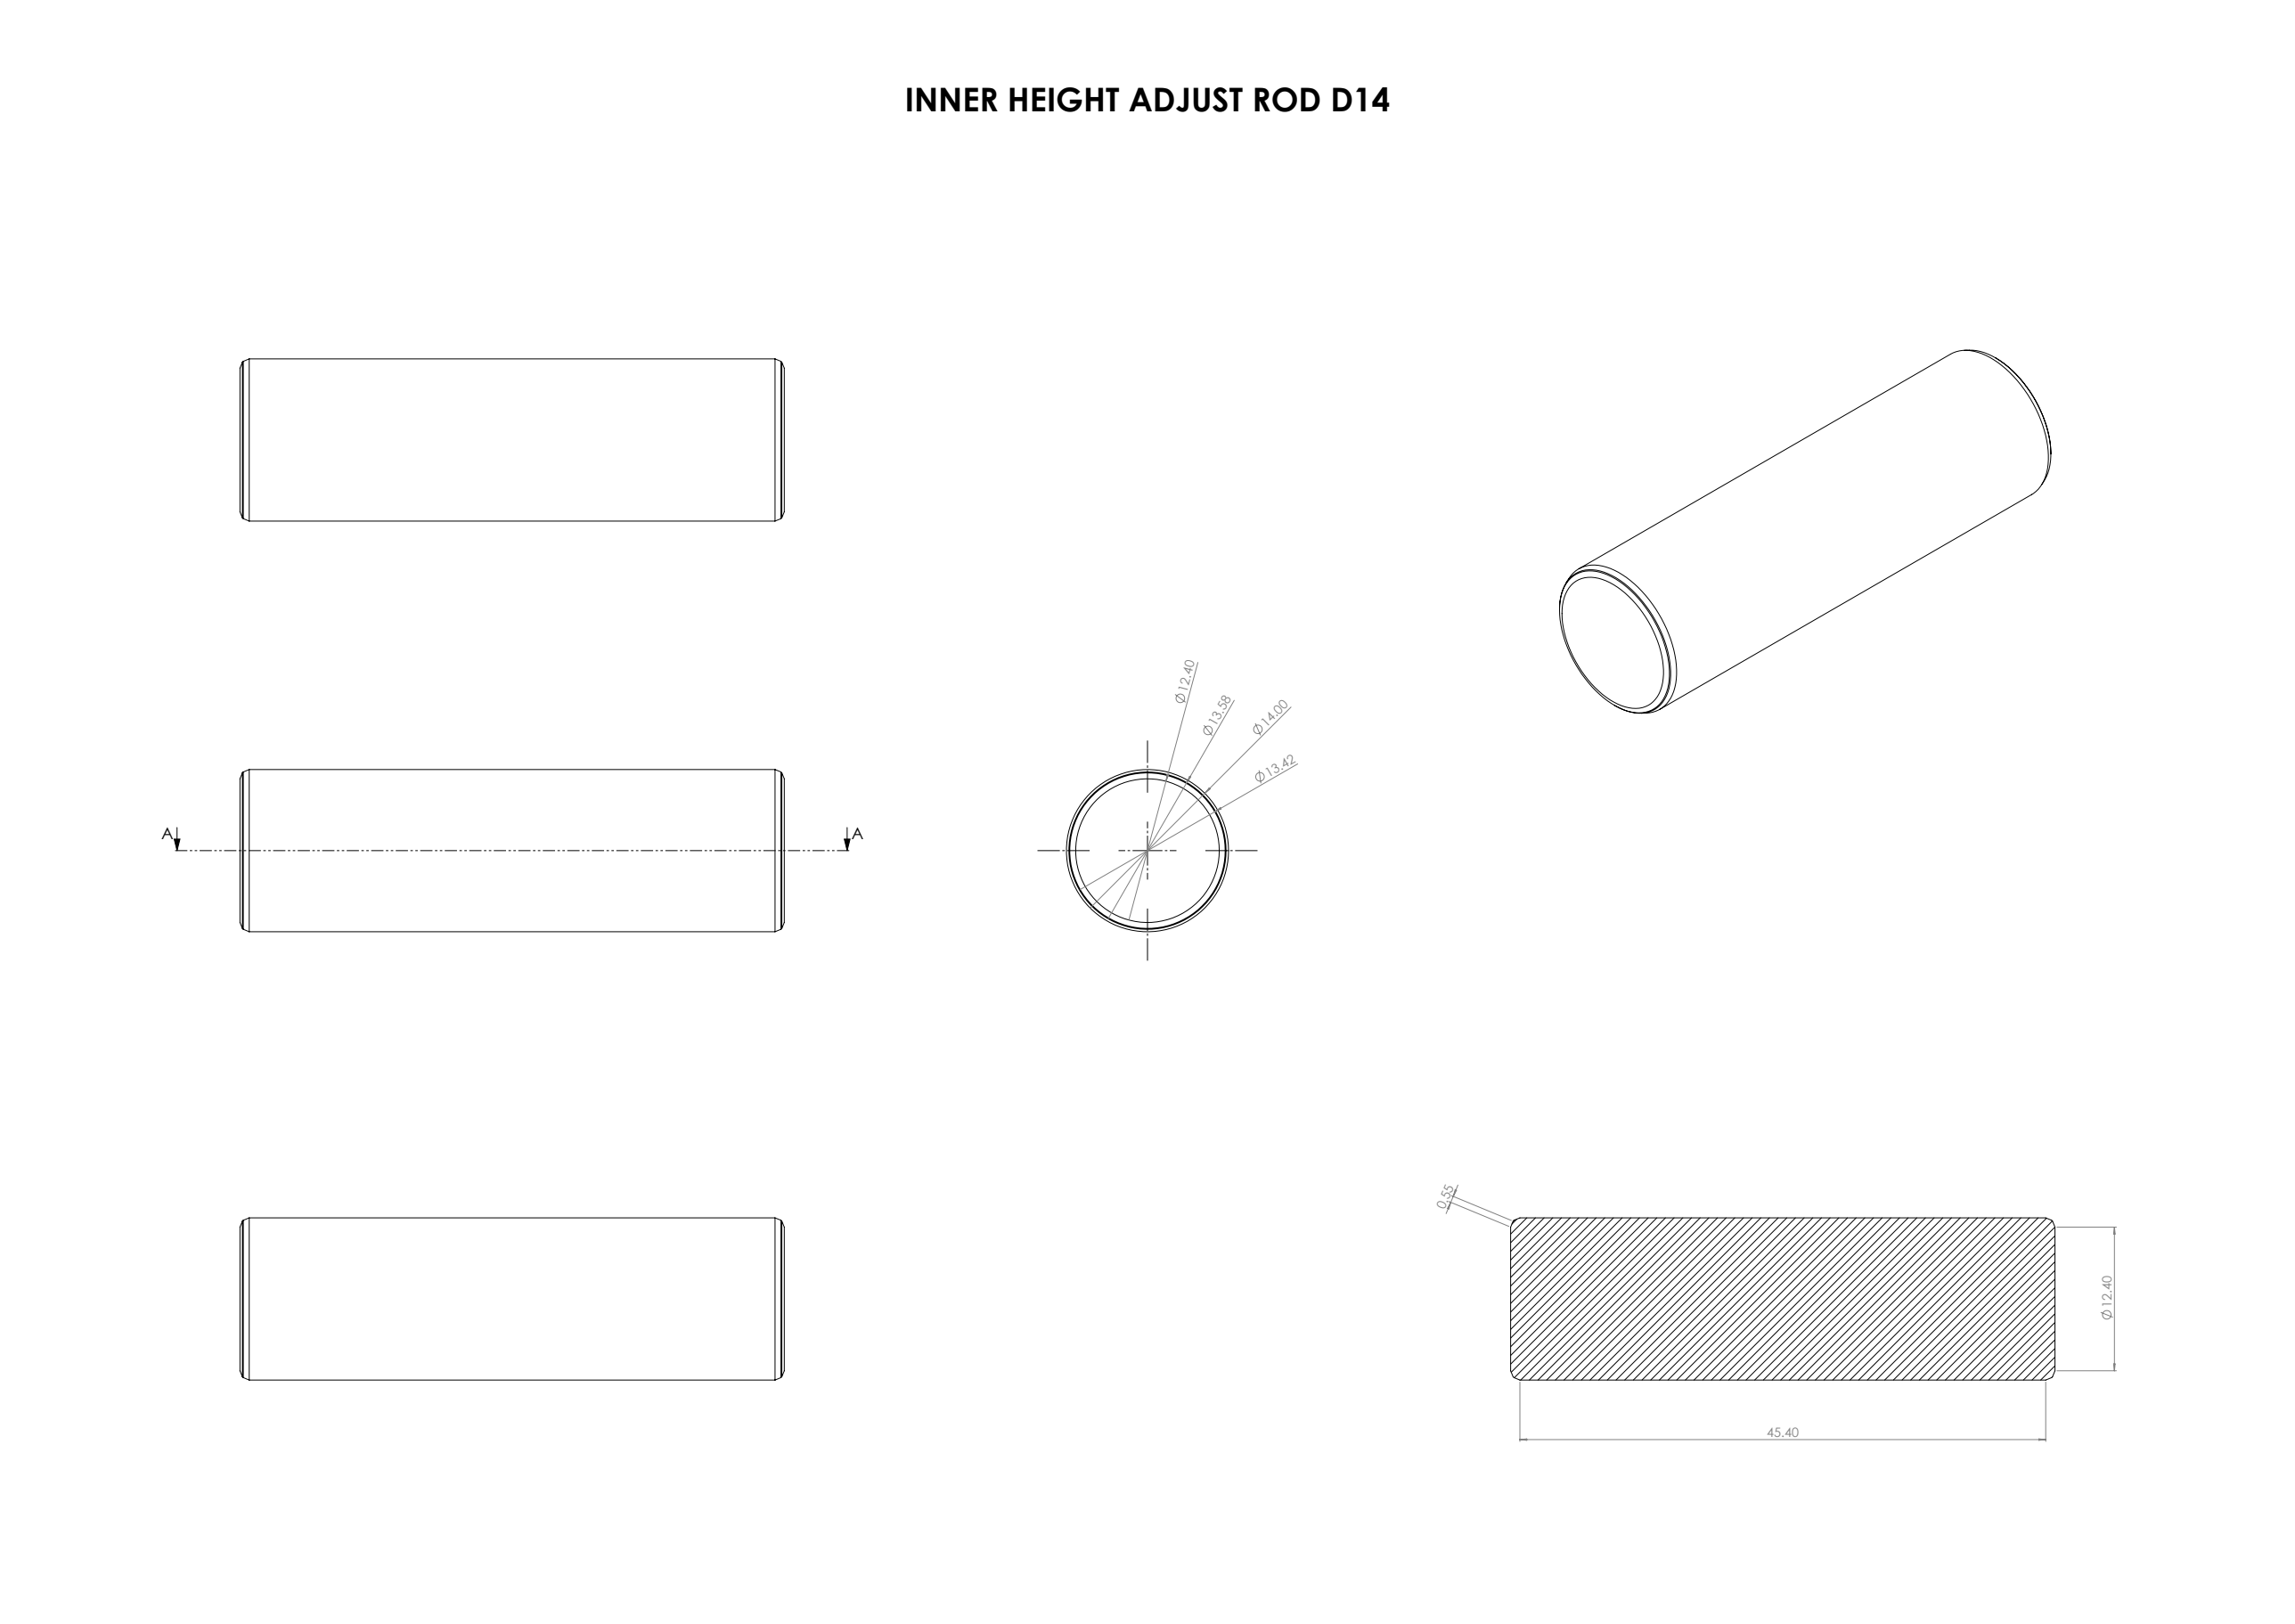
ISO-10303-21;
HEADER;
/* Generated by software containing ST-Developer
 * from STEP Tools, Inc. (www.steptools.com) 
 */

FILE_DESCRIPTION(
/* description */ (''),
/* implementation_level */ '2;1');

FILE_NAME(
/* name */ 
'03_Inner_Height_Adjust_Rod_D14.step',
/* time_stamp */ '2026-10-20T10:06:23-07:00',
/* author */ (''),
/* organization */ (''),
/* preprocessor_version */ 'ST-DEVELOPER v20.2',
/* originating_system */ 'Autodesk Translation Framework v15.15.0.0',
/* authorisation */ '');

FILE_SCHEMA (('AUTOMOTIVE_DESIGN { 1 0 10303 214 3 1 1 }'));
ENDSEC;

DATA;
#10=MECHANICAL_DESIGN_GEOMETRIC_PRESENTATION_REPRESENTATION('',(#462),#38611);
#434=SHAPE_REPRESENTATION_RELATIONSHIP('SRR','None',#38670,#448);
#448=ADVANCED_BREP_SHAPE_REPRESENTATION('',(#476),#38599);
#462=STYLED_ITEM('',(#38878),#476);
#476=MANIFOLD_SOLID_BREP('Rod',#16236);
#895=CYLINDRICAL_SURFACE('',#16637,0.7);
#1279=CIRCLE('',#16627,0.619999999999999);
#1280=CIRCLE('',#16628,0.671213203435596);
#1281=CIRCLE('',#16629,0.671213203435596);
#1282=CIRCLE('',#16631,0.678786796564404);
#1283=CIRCLE('',#16632,0.678786796564404);
#1284=CIRCLE('',#16635,0.7);
#1285=CIRCLE('',#16636,0.7);
#1286=CIRCLE('',#16638,0.7);
#1287=CIRCLE('',#16639,0.7);
#1288=CIRCLE('',#16641,0.678786796564404);
#1289=CIRCLE('',#16642,0.678786796564404);
#1290=CIRCLE('',#16644,0.671213203435597);
#1291=CIRCLE('',#16645,0.671213203435597);
#1292=CIRCLE('',#16647,0.62);
#1709=CONICAL_SURFACE('',#16626,0.645606601717798,1.17809724509618);
#1710=CONICAL_SURFACE('',#16630,0.675,0.78539816339745);
#1711=CONICAL_SURFACE('',#16634,0.689393398282202,0.392699081698726);
#1712=CONICAL_SURFACE('',#16640,0.689393398282202,0.392699081698718);
#1713=CONICAL_SURFACE('',#16643,0.675,0.785398163397447);
#1714=CONICAL_SURFACE('',#16646,0.645606601717798,1.17809724509617);
#1921=FACE_OUTER_BOUND('',#2848,.T.);
#1922=FACE_OUTER_BOUND('',#2849,.T.);
#1923=FACE_OUTER_BOUND('',#2850,.T.);
#1924=FACE_OUTER_BOUND('',#2851,.T.);
#1925=FACE_OUTER_BOUND('',#2852,.T.);
#1926=FACE_OUTER_BOUND('',#2853,.T.);
#1927=FACE_OUTER_BOUND('',#2854,.T.);
#1928=FACE_OUTER_BOUND('',#2855,.T.);
#1929=FACE_OUTER_BOUND('',#2856,.T.);
#2848=EDGE_LOOP('',(#10711,#10712,#10713,#10714,#10715));
#2849=EDGE_LOOP('',(#10716,#10717,#10718,#10719,#10720,#10721));
#2850=EDGE_LOOP('',(#10722));
#2851=EDGE_LOOP('',(#10723,#10724,#10725,#10726,#10727,#10728));
#2852=EDGE_LOOP('',(#10729,#10730,#10731,#10732,#10733,#10734));
#2853=EDGE_LOOP('',(#10735,#10736,#10737,#10738,#10739,#10740));
#2854=EDGE_LOOP('',(#10741,#10742,#10743,#10744,#10745,#10746));
#2855=EDGE_LOOP('',(#10747,#10748,#10749,#10750,#10751));
#2856=EDGE_LOOP('',(#10752));
#3908=LINE('',#22921,#5132);
#3909=LINE('',#22927,#5133);
#3910=LINE('',#22934,#5134);
#3911=LINE('',#22940,#5135);
#3912=LINE('',#22946,#5136);
#3913=LINE('',#22952,#5137);
#3914=LINE('',#22958,#5138);
#5132=VECTOR('',#18509,0.645606601717798);
#5133=VECTOR('',#18516,0.675);
#5134=VECTOR('',#18525,0.689393398282202);
#5135=VECTOR('',#18532,0.7);
#5136=VECTOR('',#18539,0.689393398282202);
#5137=VECTOR('',#18546,0.675);
#5138=VECTOR('',#18553,0.645606601717798);
#6309=VERTEX_POINT('',#22918);
#6310=VERTEX_POINT('',#22920);
#6311=VERTEX_POINT('',#22922);
#6312=VERTEX_POINT('',#22926);
#6313=VERTEX_POINT('',#22928);
#6314=VERTEX_POINT('',#22933);
#6315=VERTEX_POINT('',#22935);
#6316=VERTEX_POINT('',#22939);
#6317=VERTEX_POINT('',#22941);
#6318=VERTEX_POINT('',#22945);
#6319=VERTEX_POINT('',#22947);
#6320=VERTEX_POINT('',#22951);
#6321=VERTEX_POINT('',#22953);
#6322=VERTEX_POINT('',#22957);
#7971=EDGE_CURVE('',#6309,#6309,#1279,.T.);
#7972=EDGE_CURVE('',#6309,#6310,#3908,.T.);
#7973=EDGE_CURVE('',#6310,#6311,#1280,.T.);
#7974=EDGE_CURVE('',#6311,#6310,#1281,.T.);
#7975=EDGE_CURVE('',#6311,#6312,#3909,.T.);
#7976=EDGE_CURVE('',#6313,#6312,#1282,.T.);
#7977=EDGE_CURVE('',#6312,#6313,#1283,.T.);
#7978=EDGE_CURVE('',#6313,#6314,#3910,.T.);
#7979=EDGE_CURVE('',#6314,#6315,#1284,.T.);
#7980=EDGE_CURVE('',#6315,#6314,#1285,.T.);
#7981=EDGE_CURVE('',#6315,#6316,#3911,.T.);
#7982=EDGE_CURVE('',#6317,#6316,#1286,.T.);
#7983=EDGE_CURVE('',#6316,#6317,#1287,.T.);
#7984=EDGE_CURVE('',#6317,#6318,#3912,.T.);
#7985=EDGE_CURVE('',#6318,#6319,#1288,.T.);
#7986=EDGE_CURVE('',#6319,#6318,#1289,.T.);
#7987=EDGE_CURVE('',#6319,#6320,#3913,.T.);
#7988=EDGE_CURVE('',#6321,#6320,#1290,.T.);
#7989=EDGE_CURVE('',#6320,#6321,#1291,.T.);
#7990=EDGE_CURVE('',#6321,#6322,#3914,.T.);
#7991=EDGE_CURVE('',#6322,#6322,#1292,.T.);
#10711=ORIENTED_EDGE('',*,*,#7971,.T.);
#10712=ORIENTED_EDGE('',*,*,#7972,.T.);
#10713=ORIENTED_EDGE('',*,*,#7973,.T.);
#10714=ORIENTED_EDGE('',*,*,#7974,.T.);
#10715=ORIENTED_EDGE('',*,*,#7972,.F.);
#10716=ORIENTED_EDGE('',*,*,#7973,.F.);
#10717=ORIENTED_EDGE('',*,*,#7974,.F.);
#10718=ORIENTED_EDGE('',*,*,#7975,.T.);
#10719=ORIENTED_EDGE('',*,*,#7976,.F.);
#10720=ORIENTED_EDGE('',*,*,#7977,.F.);
#10721=ORIENTED_EDGE('',*,*,#7975,.F.);
#10722=ORIENTED_EDGE('',*,*,#7971,.F.);
#10723=ORIENTED_EDGE('',*,*,#7976,.T.);
#10724=ORIENTED_EDGE('',*,*,#7977,.T.);
#10725=ORIENTED_EDGE('',*,*,#7978,.T.);
#10726=ORIENTED_EDGE('',*,*,#7979,.T.);
#10727=ORIENTED_EDGE('',*,*,#7980,.T.);
#10728=ORIENTED_EDGE('',*,*,#7978,.F.);
#10729=ORIENTED_EDGE('',*,*,#7979,.F.);
#10730=ORIENTED_EDGE('',*,*,#7980,.F.);
#10731=ORIENTED_EDGE('',*,*,#7981,.T.);
#10732=ORIENTED_EDGE('',*,*,#7982,.F.);
#10733=ORIENTED_EDGE('',*,*,#7983,.F.);
#10734=ORIENTED_EDGE('',*,*,#7981,.F.);
#10735=ORIENTED_EDGE('',*,*,#7982,.T.);
#10736=ORIENTED_EDGE('',*,*,#7983,.T.);
#10737=ORIENTED_EDGE('',*,*,#7984,.T.);
#10738=ORIENTED_EDGE('',*,*,#7985,.T.);
#10739=ORIENTED_EDGE('',*,*,#7986,.T.);
#10740=ORIENTED_EDGE('',*,*,#7984,.F.);
#10741=ORIENTED_EDGE('',*,*,#7985,.F.);
#10742=ORIENTED_EDGE('',*,*,#7986,.F.);
#10743=ORIENTED_EDGE('',*,*,#7987,.T.);
#10744=ORIENTED_EDGE('',*,*,#7988,.F.);
#10745=ORIENTED_EDGE('',*,*,#7989,.F.);
#10746=ORIENTED_EDGE('',*,*,#7987,.F.);
#10747=ORIENTED_EDGE('',*,*,#7988,.T.);
#10748=ORIENTED_EDGE('',*,*,#7989,.T.);
#10749=ORIENTED_EDGE('',*,*,#7990,.T.);
#10750=ORIENTED_EDGE('',*,*,#7991,.T.);
#10751=ORIENTED_EDGE('',*,*,#7990,.F.);
#10752=ORIENTED_EDGE('',*,*,#7991,.F.);
#14896=PLANE('',#16633);
#14897=PLANE('',#16648);
#15464=ADVANCED_FACE('',(#1921),#1709,.T.);
#15465=ADVANCED_FACE('',(#1922),#1710,.T.);
#15466=ADVANCED_FACE('',(#1923),#14896,.T.);
#15467=ADVANCED_FACE('',(#1924),#1711,.T.);
#15468=ADVANCED_FACE('',(#1925),#895,.T.);
#15469=ADVANCED_FACE('',(#1926),#1712,.T.);
#15470=ADVANCED_FACE('',(#1927),#1713,.T.);
#15471=ADVANCED_FACE('',(#1928),#1714,.T.);
#15472=ADVANCED_FACE('',(#1929),#14897,.T.);
#16236=CLOSED_SHELL('',(#15464,#15465,#15466,#15467,#15468,#15469,#15470,
#15471,#15472));
#16625=AXIS2_PLACEMENT_3D('',#22916,#18503,#18504);
#16626=AXIS2_PLACEMENT_3D('',#22917,#18505,#18506);
#16627=AXIS2_PLACEMENT_3D('',#22919,#18507,#18508);
#16628=AXIS2_PLACEMENT_3D('',#22923,#18510,#18511);
#16629=AXIS2_PLACEMENT_3D('',#22924,#18512,#18513);
#16630=AXIS2_PLACEMENT_3D('',#22925,#18514,#18515);
#16631=AXIS2_PLACEMENT_3D('',#22929,#18517,#18518);
#16632=AXIS2_PLACEMENT_3D('',#22930,#18519,#18520);
#16633=AXIS2_PLACEMENT_3D('',#22931,#18521,#18522);
#16634=AXIS2_PLACEMENT_3D('',#22932,#18523,#18524);
#16635=AXIS2_PLACEMENT_3D('',#22936,#18526,#18527);
#16636=AXIS2_PLACEMENT_3D('',#22937,#18528,#18529);
#16637=AXIS2_PLACEMENT_3D('',#22938,#18530,#18531);
#16638=AXIS2_PLACEMENT_3D('',#22942,#18533,#18534);
#16639=AXIS2_PLACEMENT_3D('',#22943,#18535,#18536);
#16640=AXIS2_PLACEMENT_3D('',#22944,#18537,#18538);
#16641=AXIS2_PLACEMENT_3D('',#22948,#18540,#18541);
#16642=AXIS2_PLACEMENT_3D('',#22949,#18542,#18543);
#16643=AXIS2_PLACEMENT_3D('',#22950,#18544,#18545);
#16644=AXIS2_PLACEMENT_3D('',#22954,#18547,#18548);
#16645=AXIS2_PLACEMENT_3D('',#22955,#18549,#18550);
#16646=AXIS2_PLACEMENT_3D('',#22956,#18551,#18552);
#16647=AXIS2_PLACEMENT_3D('',#22959,#18554,#18555);
#16648=AXIS2_PLACEMENT_3D('',#22960,#18556,#18557);
#18503=DIRECTION('axis',(0.,0.,1.));
#18504=DIRECTION('refdir',(1.,0.,0.));
#18505=DIRECTION('center_axis',(0.,-1.93747046180099E-15,-1.));
#18506=DIRECTION('ref_axis',(-1.,-3.18304947217744E-17,0.));
#18507=DIRECTION('center_axis',(0.,0.,-1.));
#18508=DIRECTION('ref_axis',(-1.,0.,0.));
#18509=DIRECTION('',(0.923879532511291,-5.98887692616032E-16,-0.38268343236508));
#18510=DIRECTION('center_axis',(0.,0.,1.));
#18511=DIRECTION('ref_axis',(-1.,-6.12323399573677E-17,0.));
#18512=DIRECTION('center_axis',(0.,0.,1.));
#18513=DIRECTION('ref_axis',(-1.,-6.12323399573677E-17,0.));
#18514=DIRECTION('center_axis',(0.,0.,-1.));
#18515=DIRECTION('ref_axis',(1.,0.,0.));
#18516=DIRECTION('',(-0.707106781186548,-8.65956056235494E-17,-0.707106781186547));
#18517=DIRECTION('center_axis',(0.,0.,-1.));
#18518=DIRECTION('ref_axis',(-1.,-6.12323399573677E-17,0.));
#18519=DIRECTION('center_axis',(0.,0.,-1.));
#18520=DIRECTION('ref_axis',(-1.,-6.12323399573677E-17,0.));
#18521=DIRECTION('center_axis',(0.,0.,1.));
#18522=DIRECTION('ref_axis',(1.,0.,0.));
#18523=DIRECTION('center_axis',(0.,8.11581801128163E-16,-1.));
#18524=DIRECTION('ref_axis',(-1.,-3.01451275783686E-17,0.));
#18525=DIRECTION('',(0.382683432365092,8.08205059964992E-16,-0.923879532511286));
#18526=DIRECTION('center_axis',(0.,0.,1.));
#18527=DIRECTION('ref_axis',(-1.,0.,0.));
#18528=DIRECTION('center_axis',(0.,0.,1.));
#18529=DIRECTION('ref_axis',(-1.,0.,0.));
#18530=DIRECTION('center_axis',(0.,0.,1.));
#18531=DIRECTION('ref_axis',(1.,0.,0.));
#18532=DIRECTION('',(0.,0.,-1.));
#18533=DIRECTION('center_axis',(0.,0.,-1.));
#18534=DIRECTION('ref_axis',(-1.,0.,0.));
#18535=DIRECTION('center_axis',(0.,0.,-1.));
#18536=DIRECTION('ref_axis',(-1.,0.,0.));
#18537=DIRECTION('center_axis',(0.,8.11581801128149E-16,1.));
#18538=DIRECTION('ref_axis',(-1.,-3.01451275783686E-17,0.));
#18539=DIRECTION('',(-0.382683432365084,-8.0820505996498E-16,-0.923879532511289));
#18540=DIRECTION('center_axis',(0.,0.,1.));
#18541=DIRECTION('ref_axis',(-1.,-6.12323399573677E-17,0.));
#18542=DIRECTION('center_axis',(0.,0.,1.));
#18543=DIRECTION('ref_axis',(-1.,-6.12323399573677E-17,0.));
#18544=DIRECTION('center_axis',(0.,0.,1.));
#18545=DIRECTION('ref_axis',(1.,0.,0.));
#18546=DIRECTION('',(0.707106781186547,8.65956056235492E-17,-0.707106781186548));
#18547=DIRECTION('center_axis',(0.,0.,-1.));
#18548=DIRECTION('ref_axis',(-1.,-6.12323399573676E-17,0.));
#18549=DIRECTION('center_axis',(0.,0.,-1.));
#18550=DIRECTION('ref_axis',(-1.,-6.12323399573676E-17,0.));
#18551=DIRECTION('center_axis',(0.,-1.93747046180093E-15,1.));
#18552=DIRECTION('ref_axis',(-1.,-3.18304947217744E-17,0.));
#18553=DIRECTION('',(-0.923879532511287,5.98887692616029E-16,-0.38268343236509));
#18554=DIRECTION('center_axis',(0.,0.,1.));
#18555=DIRECTION('ref_axis',(-1.,0.,0.));
#18556=DIRECTION('center_axis',(0.,0.,-1.));
#18557=DIRECTION('ref_axis',(-1.,0.,0.));
#22916=CARTESIAN_POINT('',(0.,0.,0.));
#22917=CARTESIAN_POINT('Origin',(0.,-2.05499775283211E-17,6.0893933982822));
#22918=CARTESIAN_POINT('',(0.619999999999999,-7.59281015471358E-17,6.1));
#22919=CARTESIAN_POINT('Origin',(0.,0.,6.1));
#22920=CARTESIAN_POINT('',(0.671213203435596,8.21999101132844E-17,6.0787867965644));
#22921=CARTESIAN_POINT('',(0.645606601717798,7.90640058302101E-17,6.0893933982822));
#22922=CARTESIAN_POINT('',(-0.671213203435596,-8.21999101132843E-17,6.0787867965644));
#22923=CARTESIAN_POINT('Origin',(0.,-4.10999550566422E-17,6.0787867965644));
#22924=CARTESIAN_POINT('Origin',(0.,-4.10999550566422E-17,6.0787867965644));
#22925=CARTESIAN_POINT('Origin',(0.,0.,6.075));
#22926=CARTESIAN_POINT('',(-0.678786796564404,-8.31274077716083E-17,6.0712132034356));
#22927=CARTESIAN_POINT('',(-0.675,-8.26636589424463E-17,6.075));
#22928=CARTESIAN_POINT('',(0.678786796564404,-8.31274077716082E-17,6.0712132034356));
#22929=CARTESIAN_POINT('Origin',(0.,-4.15637038858041E-17,6.0712132034356));
#22930=CARTESIAN_POINT('Origin',(0.,-4.15637038858041E-17,6.0712132034356));
#22931=CARTESIAN_POINT('Origin',(0.,0.,6.1));
#22932=CARTESIAN_POINT('Origin',(0.,-2.07818519429021E-17,6.0456066017178));
#22933=CARTESIAN_POINT('',(0.7,8.57252759403147E-17,6.02));
#22934=CARTESIAN_POINT('',(0.689393398282202,8.44263418559615E-17,6.0456066017178));
#22935=CARTESIAN_POINT('',(-0.7,-8.57252759403147E-17,6.02));
#22936=CARTESIAN_POINT('Origin',(0.,0.,6.02));
#22937=CARTESIAN_POINT('Origin',(0.,0.,6.02));
#22938=CARTESIAN_POINT('Origin',(0.,0.,3.75));
#22939=CARTESIAN_POINT('',(-0.7,-8.57252759403147E-17,1.48));
#22940=CARTESIAN_POINT('',(-0.7,-8.57252759403147E-17,3.75));
#22941=CARTESIAN_POINT('',(0.7,-8.57252759403147E-17,1.48));
#22942=CARTESIAN_POINT('Origin',(0.,0.,1.48));
#22943=CARTESIAN_POINT('Origin',(0.,0.,1.48));
#22944=CARTESIAN_POINT('Origin',(0.,-2.07818519429021E-17,1.4543933982822));
#22945=CARTESIAN_POINT('',(0.678786796564404,8.31274077716083E-17,1.4287867965644));
#22946=CARTESIAN_POINT('',(0.689393398282202,8.44263418559615E-17,1.4543933982822));
#22947=CARTESIAN_POINT('',(-0.678786796564404,-8.31274077716083E-17,1.4287867965644));
#22948=CARTESIAN_POINT('Origin',(0.,-4.15637038858041E-17,1.4287867965644));
#22949=CARTESIAN_POINT('Origin',(0.,-4.15637038858041E-17,1.4287867965644));
#22950=CARTESIAN_POINT('Origin',(0.,0.,1.425));
#22951=CARTESIAN_POINT('',(-0.671213203435597,-8.21999101132845E-17,1.4212132034356));
#22952=CARTESIAN_POINT('',(-0.675,-8.26636589424463E-17,1.425));
#22953=CARTESIAN_POINT('',(0.671213203435597,-8.21999101132845E-17,1.4212132034356));
#22954=CARTESIAN_POINT('Origin',(0.,-4.10999550566422E-17,1.4212132034356));
#22955=CARTESIAN_POINT('Origin',(0.,-4.10999550566422E-17,1.4212132034356));
#22956=CARTESIAN_POINT('Origin',(0.,-2.05499775283211E-17,1.4106066017178));
#22957=CARTESIAN_POINT('',(0.62,7.59281015471359E-17,1.4));
#22958=CARTESIAN_POINT('',(0.645606601717798,7.90640058302102E-17,1.4106066017178));
#22959=CARTESIAN_POINT('Origin',(0.,0.,1.4));
#22960=CARTESIAN_POINT('Origin',(0.65,0.,1.4));
#38583=UNCERTAINTY_MEASURE_WITH_UNIT(LENGTH_MEASURE(0.001),#38612,
'DISTANCE_ACCURACY_VALUE',
'Maximum model space distance between geometric entities at asserted c
onnectivities');
#38595=UNCERTAINTY_MEASURE_WITH_UNIT(LENGTH_MEASURE(0.001),#38612,
'DISTANCE_ACCURACY_VALUE',
'Maximum model space distance between geometric entities at asserted c
onnectivities');
#38599=(
GEOMETRIC_REPRESENTATION_CONTEXT(3)
GLOBAL_UNCERTAINTY_ASSIGNED_CONTEXT((#38583))
GLOBAL_UNIT_ASSIGNED_CONTEXT((#38612,#38614,#38615))
REPRESENTATION_CONTEXT('','3D')
);
#38611=(
GEOMETRIC_REPRESENTATION_CONTEXT(3)
GLOBAL_UNCERTAINTY_ASSIGNED_CONTEXT((#38595))
GLOBAL_UNIT_ASSIGNED_CONTEXT((#38612,#38614,#38615))
REPRESENTATION_CONTEXT('','3D')
);
#38612=(
LENGTH_UNIT()
NAMED_UNIT(*)
SI_UNIT(.CENTI.,.METRE.)
);
#38614=(
NAMED_UNIT(*)
PLANE_ANGLE_UNIT()
SI_UNIT($,.RADIAN.)
);
#38615=(
NAMED_UNIT(*)
SI_UNIT($,.STERADIAN.)
SOLID_ANGLE_UNIT()
);
#38619=SHAPE_DEFINITION_REPRESENTATION(#38634,#38670);
#38634=PRODUCT_DEFINITION_SHAPE('',$,#38686);
#38670=SHAPE_REPRESENTATION('',(#16625),#38599);
#38682=PRODUCT_DEFINITION_CONTEXT('part definition',#38729,'design');
#38686=PRODUCT_DEFINITION('2026-10-19-02-31-28-533',
'03_Inner_Height_Adjust_Rod_D14',#38701,#38682);
#38701=PRODUCT_DEFINITION_FORMATION('',$,#38734);
#38729=APPLICATION_CONTEXT(
'Core Data for Automotive Mechanical Design Process');
#38730=PRODUCT_CONTEXT('part definition',#38729,'mechanical');
#38734=PRODUCT('2026-10-19-02-31-28-533',
'03_Inner_Height_Adjust_Rod_D14',$,(#38730));
#38872=COLOUR_RGB('Grey',0.48,0.52,0.57);
#38873=FILL_AREA_STYLE_COLOUR('',#38872);
#38874=FILL_AREA_STYLE('',(#38873));
#38875=SURFACE_STYLE_FILL_AREA(#38874);
#38876=SURFACE_SIDE_STYLE('',(#38875));
#38877=SURFACE_STYLE_USAGE(.BOTH.,#38876);
#38878=PRESENTATION_STYLE_ASSIGNMENT((#38877));
ENDSEC;
END-ISO-10303-21;
